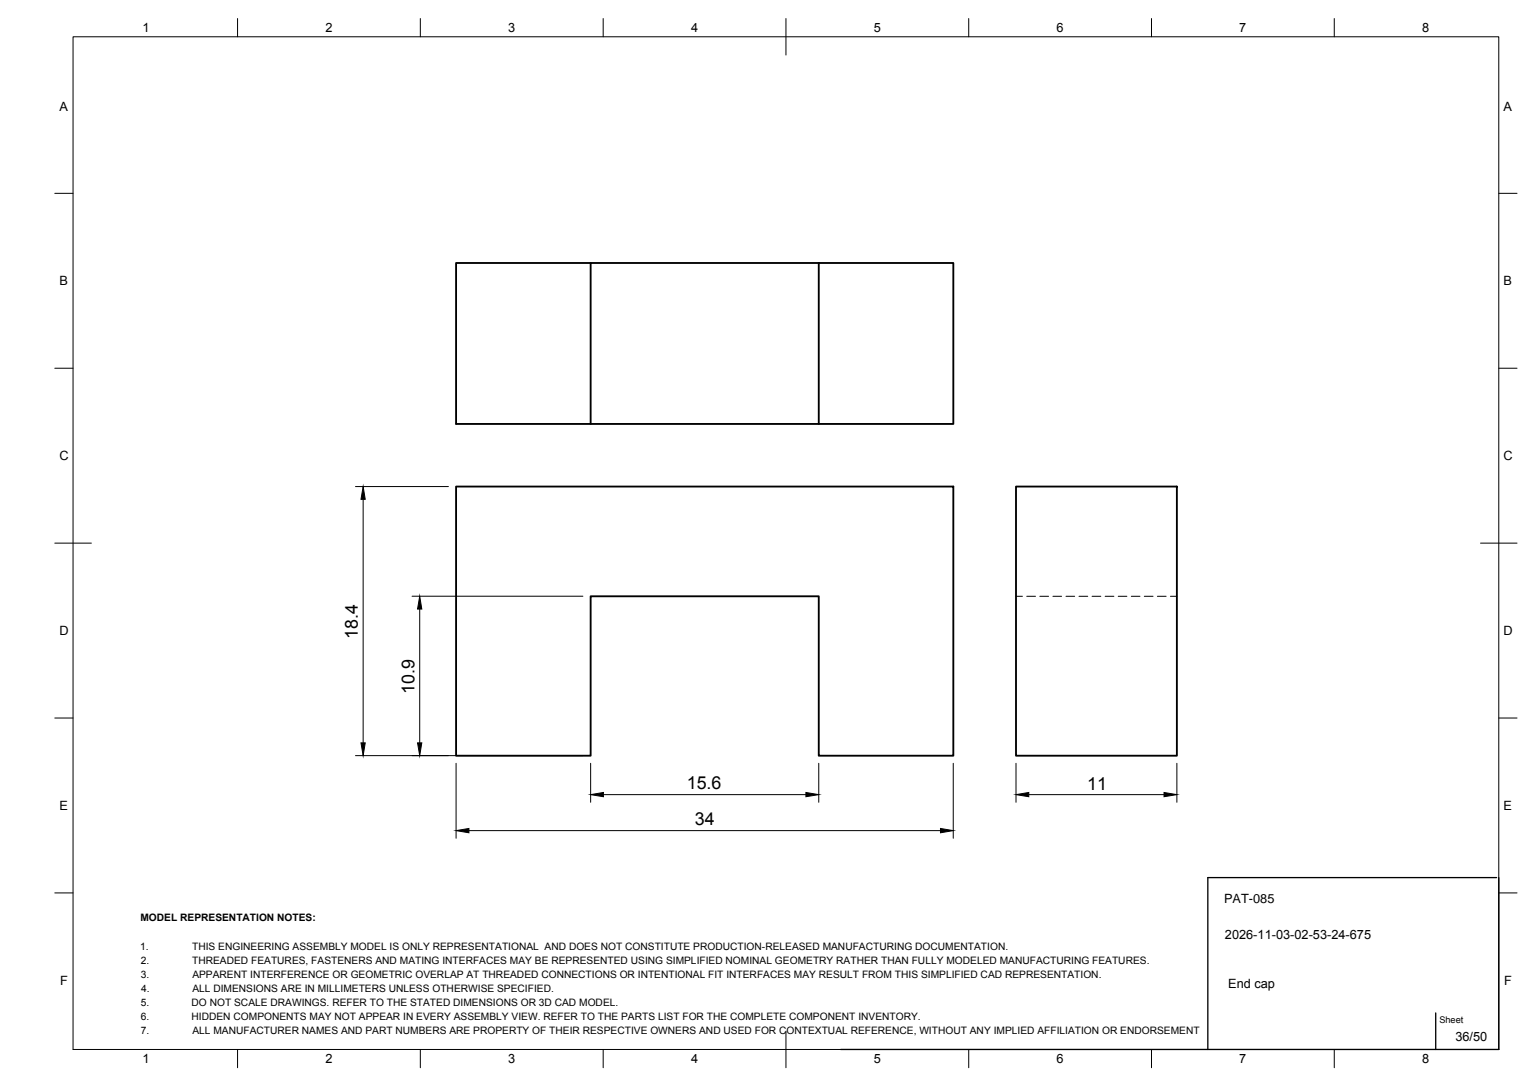
ISO-10303-21;
HEADER;
/* Generated by software containing ST-Developer
 * from STEP Tools, Inc. (www.steptools.com) 
 */

FILE_DESCRIPTION(
/* description */ ('Rack and pinion manual slide'),
/* implementation_level */ '2;1');

FILE_NAME(
/* name */ 'End cap.step',
/* time_stamp */ '2026-10-28T03:22:49-07:00',
/* author */ (''),
/* organization */ (''),
/* preprocessor_version */ 'ST-DEVELOPER v20.2',
/* originating_system */ 'Autodesk Translation Framework v15.17.0.0',
/* authorisation */ '');

FILE_SCHEMA (('AUTOMOTIVE_DESIGN { 1 0 10303 214 3 1 1 }'));
ENDSEC;

DATA;
#10=MECHANICAL_DESIGN_GEOMETRIC_PRESENTATION_REPRESENTATION('',(#768),#34851);
#669=SHAPE_REPRESENTATION_RELATIONSHIP('SRR','None',#35107,#715);
#715=ADVANCED_BREP_SHAPE_REPRESENTATION('',(#819),#34832);
#768=STYLED_ITEM('',(#35425),#819);
#819=MANIFOLD_SOLID_BREP('Body1',#13790);
#1413=PLANE('',#15161);
#1414=PLANE('',#15162);
#1415=PLANE('',#15163);
#1416=PLANE('',#15164);
#1417=PLANE('',#15165);
#1418=PLANE('',#15166);
#1419=PLANE('',#15167);
#1420=PLANE('',#15168);
#1421=PLANE('',#15169);
#1422=PLANE('',#15170);
#2046=FACE_OUTER_BOUND('',#2961,.T.);
#2047=FACE_OUTER_BOUND('',#2962,.T.);
#2048=FACE_OUTER_BOUND('',#2963,.T.);
#2049=FACE_OUTER_BOUND('',#2964,.T.);
#2050=FACE_OUTER_BOUND('',#2965,.T.);
#2051=FACE_OUTER_BOUND('',#2966,.T.);
#2052=FACE_OUTER_BOUND('',#2967,.T.);
#2053=FACE_OUTER_BOUND('',#2968,.T.);
#2054=FACE_OUTER_BOUND('',#2969,.T.);
#2055=FACE_OUTER_BOUND('',#2970,.T.);
#2961=EDGE_LOOP('',(#11804,#11805,#11806,#11807));
#2962=EDGE_LOOP('',(#11808,#11809,#11810,#11811));
#2963=EDGE_LOOP('',(#11812,#11813,#11814,#11815));
#2964=EDGE_LOOP('',(#11816,#11817,#11818,#11819));
#2965=EDGE_LOOP('',(#11820,#11821,#11822,#11823));
#2966=EDGE_LOOP('',(#11824,#11825,#11826,#11827));
#2967=EDGE_LOOP('',(#11828,#11829,#11830,#11831));
#2968=EDGE_LOOP('',(#11832,#11833,#11834,#11835));
#2969=EDGE_LOOP('',(#11836,#11837,#11838,#11839,#11840,#11841,#11842,#11843));
#2970=EDGE_LOOP('',(#11844,#11845,#11846,#11847,#11848,#11849,#11850,#11851));
#4202=LINE('',#22452,#5493);
#4203=LINE('',#22454,#5494);
#4204=LINE('',#22456,#5495);
#4205=LINE('',#22457,#5496);
#4206=LINE('',#22460,#5497);
#4207=LINE('',#22462,#5498);
#4208=LINE('',#22463,#5499);
#4209=LINE('',#22466,#5500);
#4210=LINE('',#22468,#5501);
#4211=LINE('',#22469,#5502);
#4212=LINE('',#22472,#5503);
#4213=LINE('',#22474,#5504);
#4214=LINE('',#22475,#5505);
#4215=LINE('',#22478,#5506);
#4216=LINE('',#22480,#5507);
#4217=LINE('',#22481,#5508);
#4218=LINE('',#22484,#5509);
#4219=LINE('',#22486,#5510);
#4220=LINE('',#22487,#5511);
#4221=LINE('',#22490,#5512);
#4222=LINE('',#22492,#5513);
#4223=LINE('',#22493,#5514);
#4224=LINE('',#22495,#5515);
#4225=LINE('',#22496,#5516);
#5493=VECTOR('',#18268,1.);
#5494=VECTOR('',#18269,1.);
#5495=VECTOR('',#18270,1.);
#5496=VECTOR('',#18271,1.);
#5497=VECTOR('',#18274,1.);
#5498=VECTOR('',#18275,1.);
#5499=VECTOR('',#18276,1.);
#5500=VECTOR('',#18279,1.);
#5501=VECTOR('',#18280,1.);
#5502=VECTOR('',#18281,1.);
#5503=VECTOR('',#18284,1.);
#5504=VECTOR('',#18285,1.);
#5505=VECTOR('',#18286,1.);
#5506=VECTOR('',#18289,1.);
#5507=VECTOR('',#18290,1.);
#5508=VECTOR('',#18291,1.);
#5509=VECTOR('',#18294,1.);
#5510=VECTOR('',#18295,1.);
#5511=VECTOR('',#18296,1.);
#5512=VECTOR('',#18299,1.);
#5513=VECTOR('',#18300,1.);
#5514=VECTOR('',#18301,1.);
#5515=VECTOR('',#18304,1.);
#5516=VECTOR('',#18305,1.);
#7086=VERTEX_POINT('',#22450);
#7087=VERTEX_POINT('',#22451);
#7088=VERTEX_POINT('',#22453);
#7089=VERTEX_POINT('',#22455);
#7090=VERTEX_POINT('',#22459);
#7091=VERTEX_POINT('',#22461);
#7092=VERTEX_POINT('',#22465);
#7093=VERTEX_POINT('',#22467);
#7094=VERTEX_POINT('',#22471);
#7095=VERTEX_POINT('',#22473);
#7096=VERTEX_POINT('',#22477);
#7097=VERTEX_POINT('',#22479);
#7098=VERTEX_POINT('',#22483);
#7099=VERTEX_POINT('',#22485);
#7100=VERTEX_POINT('',#22489);
#7101=VERTEX_POINT('',#22491);
#8714=EDGE_CURVE('',#7086,#7087,#4202,.T.);
#8715=EDGE_CURVE('',#7086,#7088,#4203,.T.);
#8716=EDGE_CURVE('',#7089,#7088,#4204,.T.);
#8717=EDGE_CURVE('',#7087,#7089,#4205,.T.);
#8718=EDGE_CURVE('',#7087,#7090,#4206,.T.);
#8719=EDGE_CURVE('',#7091,#7089,#4207,.T.);
#8720=EDGE_CURVE('',#7090,#7091,#4208,.T.);
#8721=EDGE_CURVE('',#7090,#7092,#4209,.T.);
#8722=EDGE_CURVE('',#7093,#7091,#4210,.T.);
#8723=EDGE_CURVE('',#7092,#7093,#4211,.T.);
#8724=EDGE_CURVE('',#7092,#7094,#4212,.T.);
#8725=EDGE_CURVE('',#7095,#7093,#4213,.T.);
#8726=EDGE_CURVE('',#7094,#7095,#4214,.T.);
#8727=EDGE_CURVE('',#7094,#7096,#4215,.T.);
#8728=EDGE_CURVE('',#7097,#7095,#4216,.T.);
#8729=EDGE_CURVE('',#7096,#7097,#4217,.T.);
#8730=EDGE_CURVE('',#7096,#7098,#4218,.T.);
#8731=EDGE_CURVE('',#7099,#7097,#4219,.T.);
#8732=EDGE_CURVE('',#7098,#7099,#4220,.T.);
#8733=EDGE_CURVE('',#7098,#7100,#4221,.T.);
#8734=EDGE_CURVE('',#7101,#7099,#4222,.T.);
#8735=EDGE_CURVE('',#7100,#7101,#4223,.T.);
#8736=EDGE_CURVE('',#7100,#7086,#4224,.T.);
#8737=EDGE_CURVE('',#7088,#7101,#4225,.T.);
#11804=ORIENTED_EDGE('',*,*,#8714,.F.);
#11805=ORIENTED_EDGE('',*,*,#8715,.T.);
#11806=ORIENTED_EDGE('',*,*,#8716,.F.);
#11807=ORIENTED_EDGE('',*,*,#8717,.F.);
#11808=ORIENTED_EDGE('',*,*,#8718,.F.);
#11809=ORIENTED_EDGE('',*,*,#8717,.T.);
#11810=ORIENTED_EDGE('',*,*,#8719,.F.);
#11811=ORIENTED_EDGE('',*,*,#8720,.F.);
#11812=ORIENTED_EDGE('',*,*,#8721,.F.);
#11813=ORIENTED_EDGE('',*,*,#8720,.T.);
#11814=ORIENTED_EDGE('',*,*,#8722,.F.);
#11815=ORIENTED_EDGE('',*,*,#8723,.F.);
#11816=ORIENTED_EDGE('',*,*,#8724,.F.);
#11817=ORIENTED_EDGE('',*,*,#8723,.T.);
#11818=ORIENTED_EDGE('',*,*,#8725,.F.);
#11819=ORIENTED_EDGE('',*,*,#8726,.F.);
#11820=ORIENTED_EDGE('',*,*,#8727,.F.);
#11821=ORIENTED_EDGE('',*,*,#8726,.T.);
#11822=ORIENTED_EDGE('',*,*,#8728,.F.);
#11823=ORIENTED_EDGE('',*,*,#8729,.F.);
#11824=ORIENTED_EDGE('',*,*,#8730,.F.);
#11825=ORIENTED_EDGE('',*,*,#8729,.T.);
#11826=ORIENTED_EDGE('',*,*,#8731,.F.);
#11827=ORIENTED_EDGE('',*,*,#8732,.F.);
#11828=ORIENTED_EDGE('',*,*,#8733,.F.);
#11829=ORIENTED_EDGE('',*,*,#8732,.T.);
#11830=ORIENTED_EDGE('',*,*,#8734,.F.);
#11831=ORIENTED_EDGE('',*,*,#8735,.F.);
#11832=ORIENTED_EDGE('',*,*,#8736,.F.);
#11833=ORIENTED_EDGE('',*,*,#8735,.T.);
#11834=ORIENTED_EDGE('',*,*,#8737,.F.);
#11835=ORIENTED_EDGE('',*,*,#8715,.F.);
#11836=ORIENTED_EDGE('',*,*,#8736,.T.);
#11837=ORIENTED_EDGE('',*,*,#8714,.T.);
#11838=ORIENTED_EDGE('',*,*,#8718,.T.);
#11839=ORIENTED_EDGE('',*,*,#8721,.T.);
#11840=ORIENTED_EDGE('',*,*,#8724,.T.);
#11841=ORIENTED_EDGE('',*,*,#8727,.T.);
#11842=ORIENTED_EDGE('',*,*,#8730,.T.);
#11843=ORIENTED_EDGE('',*,*,#8733,.T.);
#11844=ORIENTED_EDGE('',*,*,#8737,.T.);
#11845=ORIENTED_EDGE('',*,*,#8734,.T.);
#11846=ORIENTED_EDGE('',*,*,#8731,.T.);
#11847=ORIENTED_EDGE('',*,*,#8728,.T.);
#11848=ORIENTED_EDGE('',*,*,#8725,.T.);
#11849=ORIENTED_EDGE('',*,*,#8722,.T.);
#11850=ORIENTED_EDGE('',*,*,#8719,.T.);
#11851=ORIENTED_EDGE('',*,*,#8716,.T.);
#13524=ADVANCED_FACE('',(#2046),#1413,.T.);
#13525=ADVANCED_FACE('',(#2047),#1414,.T.);
#13526=ADVANCED_FACE('',(#2048),#1415,.T.);
#13527=ADVANCED_FACE('',(#2049),#1416,.T.);
#13528=ADVANCED_FACE('',(#2050),#1417,.T.);
#13529=ADVANCED_FACE('',(#2051),#1418,.T.);
#13530=ADVANCED_FACE('',(#2052),#1419,.T.);
#13531=ADVANCED_FACE('',(#2053),#1420,.T.);
#13532=ADVANCED_FACE('',(#2054),#1421,.T.);
#13533=ADVANCED_FACE('',(#2055),#1422,.T.);
#13790=CLOSED_SHELL('',(#13524,#13525,#13526,#13527,#13528,#13529,#13530,
#13531,#13532,#13533));
#15160=AXIS2_PLACEMENT_3D('',#22448,#18264,#18265);
#15161=AXIS2_PLACEMENT_3D('',#22449,#18266,#18267);
#15162=AXIS2_PLACEMENT_3D('',#22458,#18272,#18273);
#15163=AXIS2_PLACEMENT_3D('',#22464,#18277,#18278);
#15164=AXIS2_PLACEMENT_3D('',#22470,#18282,#18283);
#15165=AXIS2_PLACEMENT_3D('',#22476,#18287,#18288);
#15166=AXIS2_PLACEMENT_3D('',#22482,#18292,#18293);
#15167=AXIS2_PLACEMENT_3D('',#22488,#18297,#18298);
#15168=AXIS2_PLACEMENT_3D('',#22494,#18302,#18303);
#15169=AXIS2_PLACEMENT_3D('',#22497,#18306,#18307);
#15170=AXIS2_PLACEMENT_3D('',#22498,#18308,#18309);
#18264=DIRECTION('axis',(0.,0.,1.));
#18265=DIRECTION('refdir',(1.,0.,0.));
#18266=DIRECTION('center_axis',(0.,0.,-1.));
#18267=DIRECTION('ref_axis',(0.,-1.,0.));
#18268=DIRECTION('',(0.,1.,0.));
#18269=DIRECTION('',(-1.,0.,0.));
#18270=DIRECTION('',(0.,-1.,0.));
#18271=DIRECTION('',(-1.,0.,0.));
#18272=DIRECTION('center_axis',(0.,1.,0.));
#18273=DIRECTION('ref_axis',(0.,0.,-1.));
#18274=DIRECTION('',(0.,0.,1.));
#18275=DIRECTION('',(0.,0.,-1.));
#18276=DIRECTION('',(-1.,0.,0.));
#18277=DIRECTION('center_axis',(0.,0.,-1.));
#18278=DIRECTION('ref_axis',(0.,-1.,0.));
#18279=DIRECTION('',(0.,1.,0.));
#18280=DIRECTION('',(0.,-1.,0.));
#18281=DIRECTION('',(-1.,0.,0.));
#18282=DIRECTION('center_axis',(0.,-1.,0.));
#18283=DIRECTION('ref_axis',(0.,0.,1.));
#18284=DIRECTION('',(0.,0.,-1.));
#18285=DIRECTION('',(0.,0.,1.));
#18286=DIRECTION('',(-1.,0.,0.));
#18287=DIRECTION('center_axis',(0.,0.,-1.));
#18288=DIRECTION('ref_axis',(0.,-1.,0.));
#18289=DIRECTION('',(0.,1.,0.));
#18290=DIRECTION('',(0.,-1.,0.));
#18291=DIRECTION('',(-1.,0.,0.));
#18292=DIRECTION('center_axis',(0.,1.,0.));
#18293=DIRECTION('ref_axis',(0.,0.,-1.));
#18294=DIRECTION('',(0.,0.,1.));
#18295=DIRECTION('',(0.,0.,-1.));
#18296=DIRECTION('',(-1.,0.,0.));
#18297=DIRECTION('center_axis',(0.,0.,1.));
#18298=DIRECTION('ref_axis',(0.,1.,0.));
#18299=DIRECTION('',(0.,-1.,0.));
#18300=DIRECTION('',(0.,1.,0.));
#18301=DIRECTION('',(-1.,0.,0.));
#18302=DIRECTION('center_axis',(0.,-1.,0.));
#18303=DIRECTION('ref_axis',(0.,0.,1.));
#18304=DIRECTION('',(0.,0.,-1.));
#18305=DIRECTION('',(0.,0.,1.));
#18306=DIRECTION('center_axis',(1.,0.,0.));
#18307=DIRECTION('ref_axis',(0.,0.,-1.));
#18308=DIRECTION('center_axis',(-1.,0.,0.));
#18309=DIRECTION('ref_axis',(0.,0.,1.));
#22448=CARTESIAN_POINT('',(0.,0.,0.));
#22449=CARTESIAN_POINT('Origin',(-1.97,-0.78,0.46));
#22450=CARTESIAN_POINT('',(-1.97,-1.7,0.46));
#22451=CARTESIAN_POINT('',(-1.97,-0.78,0.46));
#22452=CARTESIAN_POINT('',(-1.97,-1.7,0.46));
#22453=CARTESIAN_POINT('',(-3.07,-1.7,0.46));
#22454=CARTESIAN_POINT('',(-1.97,-1.7,0.46));
#22455=CARTESIAN_POINT('',(-3.07,-0.78,0.46));
#22456=CARTESIAN_POINT('',(-3.07,-1.7,0.46));
#22457=CARTESIAN_POINT('',(-1.97,-0.78,0.46));
#22458=CARTESIAN_POINT('Origin',(-1.97,-0.78,1.55));
#22459=CARTESIAN_POINT('',(-1.97,-0.78,1.55));
#22460=CARTESIAN_POINT('',(-1.97,-0.78,0.46));
#22461=CARTESIAN_POINT('',(-3.07,-0.78,1.55));
#22462=CARTESIAN_POINT('',(-3.07,-0.78,0.46));
#22463=CARTESIAN_POINT('',(-1.97,-0.78,1.55));
#22464=CARTESIAN_POINT('Origin',(-1.97,0.78,1.55));
#22465=CARTESIAN_POINT('',(-1.97,0.78,1.55));
#22466=CARTESIAN_POINT('',(-1.97,-0.78,1.55));
#22467=CARTESIAN_POINT('',(-3.07,0.78,1.55));
#22468=CARTESIAN_POINT('',(-3.07,-0.78,1.55));
#22469=CARTESIAN_POINT('',(-1.97,0.78,1.55));
#22470=CARTESIAN_POINT('Origin',(-1.97,0.78,0.46));
#22471=CARTESIAN_POINT('',(-1.97,0.78,0.46));
#22472=CARTESIAN_POINT('',(-1.97,0.78,1.55));
#22473=CARTESIAN_POINT('',(-3.07,0.78,0.46));
#22474=CARTESIAN_POINT('',(-3.07,0.78,1.55));
#22475=CARTESIAN_POINT('',(-1.97,0.78,0.46));
#22476=CARTESIAN_POINT('Origin',(-1.97,1.7,0.46));
#22477=CARTESIAN_POINT('',(-1.97,1.7,0.46));
#22478=CARTESIAN_POINT('',(-1.97,0.78,0.46));
#22479=CARTESIAN_POINT('',(-3.07,1.7,0.46));
#22480=CARTESIAN_POINT('',(-3.07,0.78,0.46));
#22481=CARTESIAN_POINT('',(-1.97,1.7,0.46));
#22482=CARTESIAN_POINT('Origin',(-1.97,1.7,2.3));
#22483=CARTESIAN_POINT('',(-1.97,1.7,2.3));
#22484=CARTESIAN_POINT('',(-1.97,1.7,0.46));
#22485=CARTESIAN_POINT('',(-3.07,1.7,2.3));
#22486=CARTESIAN_POINT('',(-3.07,1.7,0.46));
#22487=CARTESIAN_POINT('',(-1.97,1.7,2.3));
#22488=CARTESIAN_POINT('Origin',(-1.97,-1.7,2.3));
#22489=CARTESIAN_POINT('',(-1.97,-1.7,2.3));
#22490=CARTESIAN_POINT('',(-1.97,1.7,2.3));
#22491=CARTESIAN_POINT('',(-3.07,-1.7,2.3));
#22492=CARTESIAN_POINT('',(-3.07,1.7,2.3));
#22493=CARTESIAN_POINT('',(-1.97,-1.7,2.3));
#22494=CARTESIAN_POINT('Origin',(-1.97,-1.7,0.46));
#22495=CARTESIAN_POINT('',(-1.97,-1.7,2.3));
#22496=CARTESIAN_POINT('',(-3.07,-1.7,2.3));
#22497=CARTESIAN_POINT('Origin',(-1.97,0.,1.38));
#22498=CARTESIAN_POINT('Origin',(-3.07,0.,1.38));
#34778=UNCERTAINTY_MEASURE_WITH_UNIT(LENGTH_MEASURE(0.001),#34852,
'DISTANCE_ACCURACY_VALUE',
'Maximum model space distance between geometric entities at asserted c
onnectivities');
#34797=UNCERTAINTY_MEASURE_WITH_UNIT(LENGTH_MEASURE(0.001),#34852,
'DISTANCE_ACCURACY_VALUE',
'Maximum model space distance between geometric entities at asserted c
onnectivities');
#34832=(
GEOMETRIC_REPRESENTATION_CONTEXT(3)
GLOBAL_UNCERTAINTY_ASSIGNED_CONTEXT((#34778))
GLOBAL_UNIT_ASSIGNED_CONTEXT((#34852,#34854,#34855))
REPRESENTATION_CONTEXT('','3D')
);
#34851=(
GEOMETRIC_REPRESENTATION_CONTEXT(3)
GLOBAL_UNCERTAINTY_ASSIGNED_CONTEXT((#34797))
GLOBAL_UNIT_ASSIGNED_CONTEXT((#34852,#34854,#34855))
REPRESENTATION_CONTEXT('','3D')
);
#34852=(
LENGTH_UNIT()
NAMED_UNIT(*)
SI_UNIT(.CENTI.,.METRE.)
);
#34854=(
NAMED_UNIT(*)
PLANE_ANGLE_UNIT()
SI_UNIT($,.RADIAN.)
);
#34855=(
NAMED_UNIT(*)
SI_UNIT($,.STERADIAN.)
SOLID_ANGLE_UNIT()
);
#34890=SHAPE_DEFINITION_REPRESENTATION(#34948,#35107);
#34948=PRODUCT_DEFINITION_SHAPE('',$,#35161);
#35107=SHAPE_REPRESENTATION('',(#15160),#34832);
#35126=PRODUCT_DEFINITION_CONTEXT('part definition',#35287,'design');
#35161=PRODUCT_DEFINITION('End cap','End cap',#35214,#35126);
#35214=PRODUCT_DEFINITION_FORMATION('',$,#35323);
#35287=APPLICATION_CONTEXT(
'Core Data for Automotive Mechanical Design Process');
#35288=PRODUCT_CONTEXT('part definition',#35287,'mechanical');
#35323=PRODUCT('End cap','End cap','End cap',(#35288));
#35419=COLOUR_RGB('Off White',0.89,0.88,0.83);
#35420=FILL_AREA_STYLE_COLOUR('',#35419);
#35421=FILL_AREA_STYLE('',(#35420));
#35422=SURFACE_STYLE_FILL_AREA(#35421);
#35423=SURFACE_SIDE_STYLE('',(#35422));
#35424=SURFACE_STYLE_USAGE(.BOTH.,#35423);
#35425=PRESENTATION_STYLE_ASSIGNMENT((#35424));
ENDSEC;
END-ISO-10303-21;
